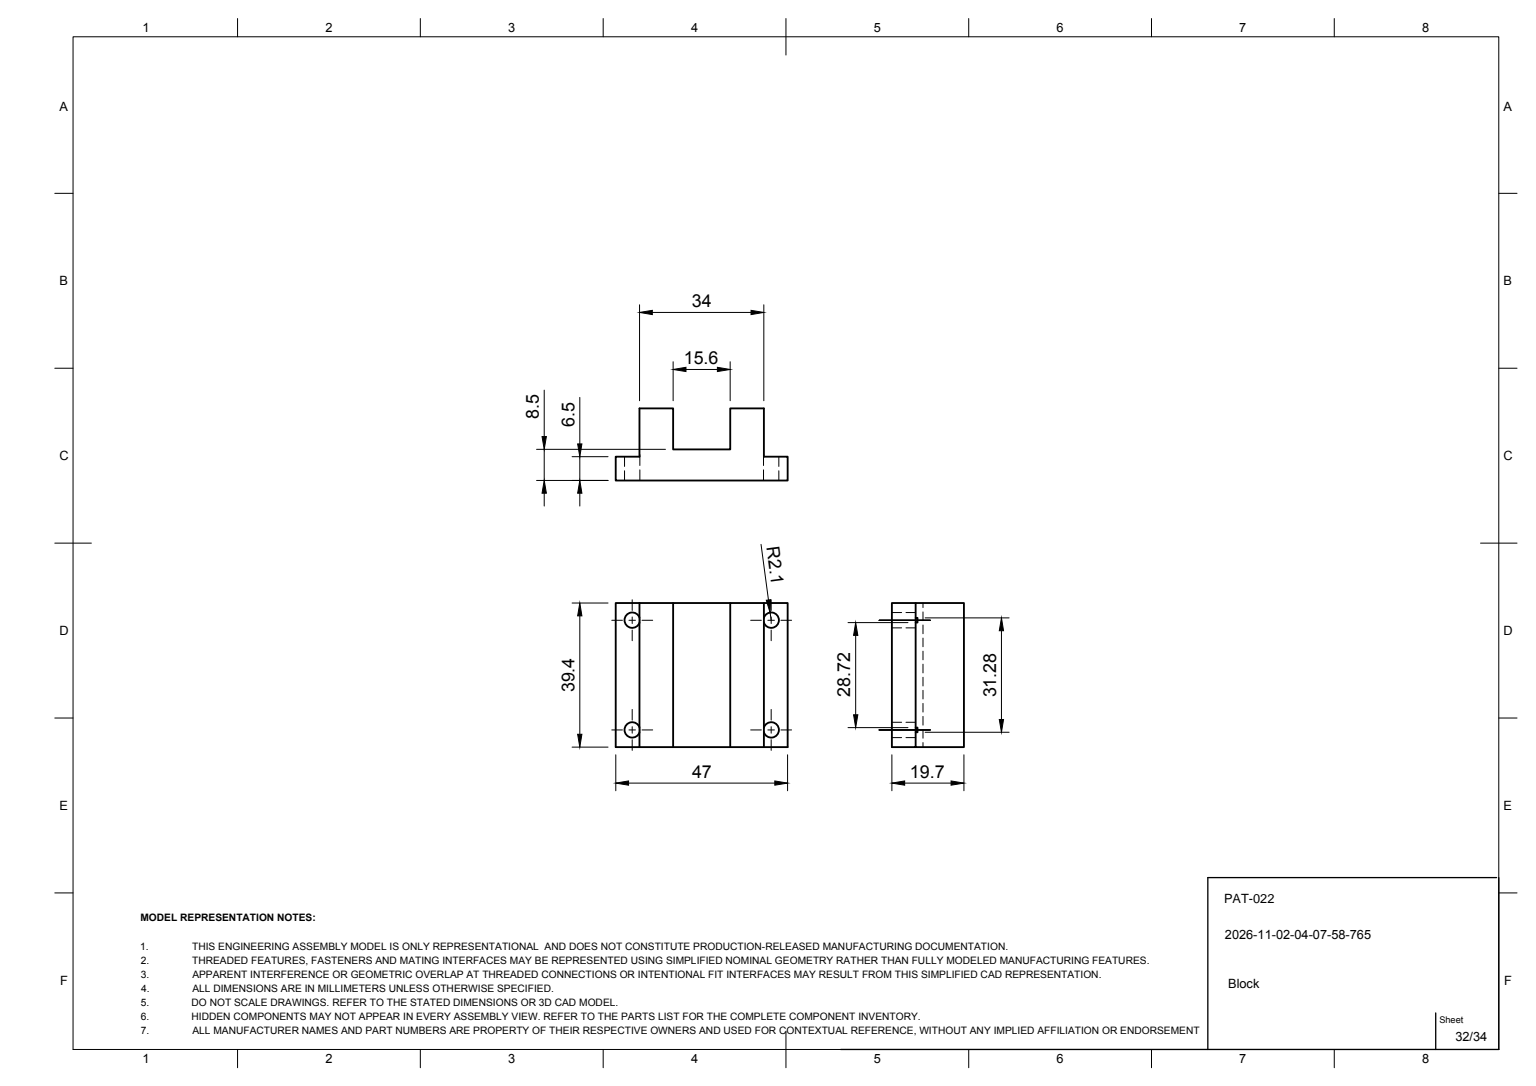
ISO-10303-21;
HEADER;
/* Generated by software containing ST-Developer
 * from STEP Tools, Inc. (www.steptools.com) 
 */

FILE_DESCRIPTION(
/* description */ ('Chute with adjustable gate'),
/* implementation_level */ '2;1');

FILE_NAME(
/* name */ 'Block.step',
/* time_stamp */ '2026-10-27T10:52:28-07:00',
/* author */ (''),
/* organization */ (''),
/* preprocessor_version */ 'ST-DEVELOPER v20.2',
/* originating_system */ 'Autodesk Translation Framework v15.17.0.0',
/* authorisation */ '');

FILE_SCHEMA (('AUTOMOTIVE_DESIGN { 1 0 10303 214 3 1 1 }'));
ENDSEC;

DATA;
#10=MECHANICAL_DESIGN_GEOMETRIC_PRESENTATION_REPRESENTATION('',(#441),#13094);
#377=SHAPE_REPRESENTATION_RELATIONSHIP('SRR','None',#13280,#409);
#409=ADVANCED_BREP_SHAPE_REPRESENTATION('',(#471),#13089);
#441=STYLED_ITEM('',(#13474),#471);
#471=MANIFOLD_SOLID_BREP('Body1',#7626);
#584=FACE_BOUND('',#1793,.T.);
#585=FACE_BOUND('',#1794,.T.);
#586=FACE_BOUND('',#1795,.T.);
#587=FACE_BOUND('',#1796,.T.);
#854=PLANE('',#8510);
#855=PLANE('',#8516);
#856=PLANE('',#8522);
#857=PLANE('',#8528);
#858=PLANE('',#8534);
#859=PLANE('',#8535);
#860=PLANE('',#8536);
#861=PLANE('',#8537);
#862=PLANE('',#8538);
#863=PLANE('',#8539);
#864=PLANE('',#8540);
#865=PLANE('',#8541);
#866=PLANE('',#8542);
#867=PLANE('',#8543);
#868=PLANE('',#8544);
#869=PLANE('',#8545);
#870=PLANE('',#8546);
#871=PLANE('',#8547);
#1254=FACE_OUTER_BOUND('',#1779,.T.);
#1255=FACE_OUTER_BOUND('',#1780,.T.);
#1256=FACE_OUTER_BOUND('',#1781,.T.);
#1257=FACE_OUTER_BOUND('',#1782,.T.);
#1258=FACE_OUTER_BOUND('',#1783,.T.);
#1259=FACE_OUTER_BOUND('',#1784,.T.);
#1260=FACE_OUTER_BOUND('',#1785,.T.);
#1261=FACE_OUTER_BOUND('',#1786,.T.);
#1262=FACE_OUTER_BOUND('',#1787,.T.);
#1263=FACE_OUTER_BOUND('',#1788,.T.);
#1264=FACE_OUTER_BOUND('',#1789,.T.);
#1265=FACE_OUTER_BOUND('',#1790,.T.);
#1266=FACE_OUTER_BOUND('',#1791,.T.);
#1267=FACE_OUTER_BOUND('',#1792,.T.);
#1268=FACE_OUTER_BOUND('',#1797,.T.);
#1269=FACE_OUTER_BOUND('',#1798,.T.);
#1270=FACE_OUTER_BOUND('',#1799,.T.);
#1271=FACE_OUTER_BOUND('',#1800,.T.);
#1272=FACE_OUTER_BOUND('',#1801,.T.);
#1273=FACE_OUTER_BOUND('',#1802,.T.);
#1274=FACE_OUTER_BOUND('',#1803,.T.);
#1275=FACE_OUTER_BOUND('',#1804,.T.);
#1779=EDGE_LOOP('',(#6742,#6743));
#1780=EDGE_LOOP('',(#6744,#6745,#6746,#6747,#6748,#6749,#6750,#6751));
#1781=EDGE_LOOP('',(#6752,#6753));
#1782=EDGE_LOOP('',(#6754,#6755,#6756,#6757,#6758,#6759,#6760,#6761));
#1783=EDGE_LOOP('',(#6762,#6763));
#1784=EDGE_LOOP('',(#6764,#6765,#6766,#6767,#6768,#6769,#6770,#6771));
#1785=EDGE_LOOP('',(#6772,#6773));
#1786=EDGE_LOOP('',(#6774,#6775,#6776,#6777,#6778,#6779,#6780,#6781));
#1787=EDGE_LOOP('',(#6782,#6783,#6784,#6785,#6786,#6787,#6788,#6789,#6790,
#6791,#6792,#6793));
#1788=EDGE_LOOP('',(#6794,#6795,#6796,#6797,#6798,#6799,#6800,#6801,#6802,
#6803,#6804,#6805));
#1789=EDGE_LOOP('',(#6806,#6807,#6808,#6809,#6810,#6811,#6812,#6813,#6814,
#6815,#6816,#6817));
#1790=EDGE_LOOP('',(#6818,#6819,#6820,#6821,#6822,#6823,#6824,#6825,#6826,
#6827));
#1791=EDGE_LOOP('',(#6828,#6829,#6830,#6831));
#1792=EDGE_LOOP('',(#6832,#6833,#6834,#6835));
#1793=EDGE_LOOP('',(#6836));
#1794=EDGE_LOOP('',(#6837));
#1795=EDGE_LOOP('',(#6838));
#1796=EDGE_LOOP('',(#6839));
#1797=EDGE_LOOP('',(#6840,#6841,#6842,#6843));
#1798=EDGE_LOOP('',(#6844,#6845,#6846,#6847,#6848,#6849,#6850,#6851,#6852,
#6853));
#1799=EDGE_LOOP('',(#6854,#6855,#6856,#6857));
#1800=EDGE_LOOP('',(#6858,#6859,#6860,#6861));
#1801=EDGE_LOOP('',(#6862,#6863,#6864,#6865));
#1802=EDGE_LOOP('',(#6866,#6867,#6868,#6869));
#1803=EDGE_LOOP('',(#6870,#6871,#6872,#6873));
#1804=EDGE_LOOP('',(#6874,#6875,#6876,#6877,#6878,#6879,#6880,#6881,#6882,
#6883,#6884,#6885));
#2486=LINE('',#12566,#3263);
#2487=LINE('',#12570,#3264);
#2488=LINE('',#12574,#3265);
#2489=LINE('',#12578,#3266);
#2490=LINE('',#12582,#3267);
#2491=LINE('',#12586,#3268);
#2492=LINE('',#12590,#3269);
#2493=LINE('',#12594,#3270);
#2494=LINE('',#12598,#3271);
#2495=LINE('',#12602,#3272);
#2496=LINE('',#12606,#3273);
#2497=LINE('',#12610,#3274);
#2498=LINE('',#12614,#3275);
#2499=LINE('',#12618,#3276);
#2500=LINE('',#12622,#3277);
#2501=LINE('',#12626,#3278);
#2502=LINE('',#12628,#3279);
#2503=LINE('',#12630,#3280);
#2504=LINE('',#12632,#3281);
#2505=LINE('',#12634,#3282);
#2506=LINE('',#12636,#3283);
#2507=LINE('',#12637,#3284);
#2508=LINE('',#12639,#3285);
#2509=LINE('',#12641,#3286);
#2510=LINE('',#12643,#3287);
#2511=LINE('',#12645,#3288);
#2512=LINE('',#12647,#3289);
#2513=LINE('',#12648,#3290);
#2514=LINE('',#12651,#3291);
#2515=LINE('',#12653,#3292);
#2516=LINE('',#12655,#3293);
#2517=LINE('',#12657,#3294);
#2518=LINE('',#12658,#3295);
#2519=LINE('',#12660,#3296);
#2520=LINE('',#12662,#3297);
#2521=LINE('',#12664,#3298);
#2522=LINE('',#12666,#3299);
#2523=LINE('',#12667,#3300);
#2524=LINE('',#12670,#3301);
#2525=LINE('',#12671,#3302);
#2526=LINE('',#12674,#3303);
#2527=LINE('',#12675,#3304);
#2528=LINE('',#12678,#3305);
#2529=LINE('',#12679,#3306);
#2530=LINE('',#12682,#3307);
#2531=LINE('',#12683,#3308);
#2532=LINE('',#12685,#3309);
#2533=LINE('',#12688,#3310);
#2534=LINE('',#12689,#3311);
#2535=LINE('',#12692,#3312);
#2536=LINE('',#12693,#3313);
#2537=LINE('',#12696,#3314);
#2538=LINE('',#12697,#3315);
#2539=LINE('',#12700,#3316);
#2540=LINE('',#12701,#3317);
#2541=LINE('',#12703,#3318);
#3263=VECTOR('',#10374,1.);
#3264=VECTOR('',#10379,1.);
#3265=VECTOR('',#10382,0.21);
#3266=VECTOR('',#10387,1.);
#3267=VECTOR('',#10390,1.);
#3268=VECTOR('',#10395,1.);
#3269=VECTOR('',#10398,0.21);
#3270=VECTOR('',#10403,1.);
#3271=VECTOR('',#10406,1.);
#3272=VECTOR('',#10411,1.);
#3273=VECTOR('',#10414,0.21);
#3274=VECTOR('',#10419,1.);
#3275=VECTOR('',#10422,1.);
#3276=VECTOR('',#10427,1.);
#3277=VECTOR('',#10430,0.21);
#3278=VECTOR('',#10435,1.);
#3279=VECTOR('',#10438,1.);
#3280=VECTOR('',#10439,1.);
#3281=VECTOR('',#10440,1.);
#3282=VECTOR('',#10441,1.);
#3283=VECTOR('',#10442,1.);
#3284=VECTOR('',#10443,1.);
#3285=VECTOR('',#10446,1.);
#3286=VECTOR('',#10447,1.);
#3287=VECTOR('',#10448,1.);
#3288=VECTOR('',#10449,1.);
#3289=VECTOR('',#10450,1.);
#3290=VECTOR('',#10451,1.);
#3291=VECTOR('',#10454,1.);
#3292=VECTOR('',#10455,1.);
#3293=VECTOR('',#10456,1.);
#3294=VECTOR('',#10457,1.);
#3295=VECTOR('',#10458,1.);
#3296=VECTOR('',#10459,1.);
#3297=VECTOR('',#10460,1.);
#3298=VECTOR('',#10461,1.);
#3299=VECTOR('',#10462,1.);
#3300=VECTOR('',#10463,1.);
#3301=VECTOR('',#10466,1.);
#3302=VECTOR('',#10467,1.);
#3303=VECTOR('',#10470,1.);
#3304=VECTOR('',#10471,1.);
#3305=VECTOR('',#10474,1.);
#3306=VECTOR('',#10475,1.);
#3307=VECTOR('',#10478,1.);
#3308=VECTOR('',#10479,1.);
#3309=VECTOR('',#10482,1.);
#3310=VECTOR('',#10485,1.);
#3311=VECTOR('',#10486,1.);
#3312=VECTOR('',#10489,1.);
#3313=VECTOR('',#10490,1.);
#3314=VECTOR('',#10493,1.);
#3315=VECTOR('',#10494,1.);
#3316=VECTOR('',#10497,1.);
#3317=VECTOR('',#10498,1.);
#3318=VECTOR('',#10501,1.);
#3562=CIRCLE('',#8511,0.21);
#3563=CIRCLE('',#8513,0.21);
#3564=CIRCLE('',#8514,0.21);
#3565=CIRCLE('',#8515,0.21);
#3566=CIRCLE('',#8517,0.21);
#3567=CIRCLE('',#8519,0.21);
#3568=CIRCLE('',#8520,0.21);
#3569=CIRCLE('',#8521,0.21);
#3570=CIRCLE('',#8523,0.21);
#3571=CIRCLE('',#8525,0.21);
#3572=CIRCLE('',#8526,0.21);
#3573=CIRCLE('',#8527,0.21);
#3574=CIRCLE('',#8529,0.21);
#3575=CIRCLE('',#8531,0.21);
#3576=CIRCLE('',#8532,0.21);
#3577=CIRCLE('',#8533,0.21);
#4107=VERTEX_POINT('',#12564);
#4108=VERTEX_POINT('',#12565);
#4109=VERTEX_POINT('',#12569);
#4110=VERTEX_POINT('',#12571);
#4111=VERTEX_POINT('',#12573);
#4112=VERTEX_POINT('',#12576);
#4113=VERTEX_POINT('',#12580);
#4114=VERTEX_POINT('',#12581);
#4115=VERTEX_POINT('',#12585);
#4116=VERTEX_POINT('',#12587);
#4117=VERTEX_POINT('',#12589);
#4118=VERTEX_POINT('',#12592);
#4119=VERTEX_POINT('',#12596);
#4120=VERTEX_POINT('',#12597);
#4121=VERTEX_POINT('',#12601);
#4122=VERTEX_POINT('',#12603);
#4123=VERTEX_POINT('',#12605);
#4124=VERTEX_POINT('',#12608);
#4125=VERTEX_POINT('',#12612);
#4126=VERTEX_POINT('',#12613);
#4127=VERTEX_POINT('',#12617);
#4128=VERTEX_POINT('',#12619);
#4129=VERTEX_POINT('',#12621);
#4130=VERTEX_POINT('',#12624);
#4131=VERTEX_POINT('',#12629);
#4132=VERTEX_POINT('',#12631);
#4133=VERTEX_POINT('',#12633);
#4134=VERTEX_POINT('',#12635);
#4135=VERTEX_POINT('',#12640);
#4136=VERTEX_POINT('',#12642);
#4137=VERTEX_POINT('',#12644);
#4138=VERTEX_POINT('',#12646);
#4139=VERTEX_POINT('',#12650);
#4140=VERTEX_POINT('',#12652);
#4141=VERTEX_POINT('',#12654);
#4142=VERTEX_POINT('',#12656);
#4143=VERTEX_POINT('',#12659);
#4144=VERTEX_POINT('',#12661);
#4145=VERTEX_POINT('',#12663);
#4146=VERTEX_POINT('',#12665);
#4147=VERTEX_POINT('',#12669);
#4148=VERTEX_POINT('',#12673);
#4149=VERTEX_POINT('',#12677);
#4150=VERTEX_POINT('',#12681);
#4151=VERTEX_POINT('',#12687);
#4152=VERTEX_POINT('',#12691);
#4153=VERTEX_POINT('',#12695);
#4154=VERTEX_POINT('',#12699);
#5004=EDGE_CURVE('',#4107,#4108,#2486,.T.);
#5005=EDGE_CURVE('',#4107,#4108,#3562,.T.);
#5006=EDGE_CURVE('',#4109,#4107,#2487,.T.);
#5007=EDGE_CURVE('',#4110,#4109,#3563,.T.);
#5008=EDGE_CURVE('',#4110,#4111,#2488,.T.);
#5009=EDGE_CURVE('',#4111,#4111,#3564,.T.);
#5010=EDGE_CURVE('',#4112,#4110,#3565,.T.);
#5011=EDGE_CURVE('',#4108,#4112,#2489,.T.);
#5012=EDGE_CURVE('',#4113,#4114,#2490,.T.);
#5013=EDGE_CURVE('',#4113,#4114,#3566,.T.);
#5014=EDGE_CURVE('',#4115,#4113,#2491,.T.);
#5015=EDGE_CURVE('',#4116,#4115,#3567,.T.);
#5016=EDGE_CURVE('',#4116,#4117,#2492,.T.);
#5017=EDGE_CURVE('',#4117,#4117,#3568,.T.);
#5018=EDGE_CURVE('',#4118,#4116,#3569,.T.);
#5019=EDGE_CURVE('',#4114,#4118,#2493,.T.);
#5020=EDGE_CURVE('',#4119,#4120,#2494,.T.);
#5021=EDGE_CURVE('',#4119,#4120,#3570,.T.);
#5022=EDGE_CURVE('',#4121,#4119,#2495,.T.);
#5023=EDGE_CURVE('',#4122,#4121,#3571,.T.);
#5024=EDGE_CURVE('',#4122,#4123,#2496,.T.);
#5025=EDGE_CURVE('',#4123,#4123,#3572,.T.);
#5026=EDGE_CURVE('',#4124,#4122,#3573,.T.);
#5027=EDGE_CURVE('',#4120,#4124,#2497,.T.);
#5028=EDGE_CURVE('',#4125,#4126,#2498,.T.);
#5029=EDGE_CURVE('',#4125,#4126,#3574,.T.);
#5030=EDGE_CURVE('',#4127,#4125,#2499,.T.);
#5031=EDGE_CURVE('',#4128,#4127,#3575,.T.);
#5032=EDGE_CURVE('',#4128,#4129,#2500,.T.);
#5033=EDGE_CURVE('',#4129,#4129,#3576,.T.);
#5034=EDGE_CURVE('',#4130,#4128,#3577,.T.);
#5035=EDGE_CURVE('',#4126,#4130,#2501,.T.);
#5036=EDGE_CURVE('',#4112,#4121,#2502,.T.);
#5037=EDGE_CURVE('',#4124,#4131,#2503,.T.);
#5038=EDGE_CURVE('',#4132,#4131,#2504,.T.);
#5039=EDGE_CURVE('',#4132,#4133,#2505,.T.);
#5040=EDGE_CURVE('',#4134,#4133,#2506,.T.);
#5041=EDGE_CURVE('',#4134,#4109,#2507,.T.);
#5042=EDGE_CURVE('',#4118,#4127,#2508,.T.);
#5043=EDGE_CURVE('',#4130,#4135,#2509,.T.);
#5044=EDGE_CURVE('',#4136,#4135,#2510,.T.);
#5045=EDGE_CURVE('',#4137,#4136,#2511,.T.);
#5046=EDGE_CURVE('',#4138,#4137,#2512,.T.);
#5047=EDGE_CURVE('',#4138,#4115,#2513,.T.);
#5048=EDGE_CURVE('',#4131,#4139,#2514,.T.);
#5049=EDGE_CURVE('',#4139,#4140,#2515,.T.);
#5050=EDGE_CURVE('',#4140,#4141,#2516,.T.);
#5051=EDGE_CURVE('',#4141,#4142,#2517,.T.);
#5052=EDGE_CURVE('',#4142,#4138,#2518,.T.);
#5053=EDGE_CURVE('',#4137,#4143,#2519,.T.);
#5054=EDGE_CURVE('',#4143,#4144,#2520,.T.);
#5055=EDGE_CURVE('',#4144,#4145,#2521,.T.);
#5056=EDGE_CURVE('',#4145,#4146,#2522,.T.);
#5057=EDGE_CURVE('',#4146,#4132,#2523,.T.);
#5058=EDGE_CURVE('',#4147,#4134,#2524,.T.);
#5059=EDGE_CURVE('',#4139,#4147,#2525,.T.);
#5060=EDGE_CURVE('',#4148,#4147,#2526,.T.);
#5061=EDGE_CURVE('',#4140,#4148,#2527,.T.);
#5062=EDGE_CURVE('',#4149,#4148,#2528,.T.);
#5063=EDGE_CURVE('',#4141,#4149,#2529,.T.);
#5064=EDGE_CURVE('',#4150,#4149,#2530,.T.);
#5065=EDGE_CURVE('',#4142,#4150,#2531,.T.);
#5066=EDGE_CURVE('',#4135,#4150,#2532,.T.);
#5067=EDGE_CURVE('',#4151,#4136,#2533,.T.);
#5068=EDGE_CURVE('',#4143,#4151,#2534,.T.);
#5069=EDGE_CURVE('',#4152,#4151,#2535,.T.);
#5070=EDGE_CURVE('',#4144,#4152,#2536,.T.);
#5071=EDGE_CURVE('',#4153,#4152,#2537,.T.);
#5072=EDGE_CURVE('',#4145,#4153,#2538,.T.);
#5073=EDGE_CURVE('',#4154,#4153,#2539,.T.);
#5074=EDGE_CURVE('',#4146,#4154,#2540,.T.);
#5075=EDGE_CURVE('',#4133,#4154,#2541,.T.);
#6742=ORIENTED_EDGE('',*,*,#5004,.F.);
#6743=ORIENTED_EDGE('',*,*,#5005,.T.);
#6744=ORIENTED_EDGE('',*,*,#5006,.F.);
#6745=ORIENTED_EDGE('',*,*,#5007,.F.);
#6746=ORIENTED_EDGE('',*,*,#5008,.T.);
#6747=ORIENTED_EDGE('',*,*,#5009,.F.);
#6748=ORIENTED_EDGE('',*,*,#5008,.F.);
#6749=ORIENTED_EDGE('',*,*,#5010,.F.);
#6750=ORIENTED_EDGE('',*,*,#5011,.F.);
#6751=ORIENTED_EDGE('',*,*,#5005,.F.);
#6752=ORIENTED_EDGE('',*,*,#5012,.F.);
#6753=ORIENTED_EDGE('',*,*,#5013,.T.);
#6754=ORIENTED_EDGE('',*,*,#5014,.F.);
#6755=ORIENTED_EDGE('',*,*,#5015,.F.);
#6756=ORIENTED_EDGE('',*,*,#5016,.T.);
#6757=ORIENTED_EDGE('',*,*,#5017,.F.);
#6758=ORIENTED_EDGE('',*,*,#5016,.F.);
#6759=ORIENTED_EDGE('',*,*,#5018,.F.);
#6760=ORIENTED_EDGE('',*,*,#5019,.F.);
#6761=ORIENTED_EDGE('',*,*,#5013,.F.);
#6762=ORIENTED_EDGE('',*,*,#5020,.F.);
#6763=ORIENTED_EDGE('',*,*,#5021,.T.);
#6764=ORIENTED_EDGE('',*,*,#5022,.F.);
#6765=ORIENTED_EDGE('',*,*,#5023,.F.);
#6766=ORIENTED_EDGE('',*,*,#5024,.T.);
#6767=ORIENTED_EDGE('',*,*,#5025,.F.);
#6768=ORIENTED_EDGE('',*,*,#5024,.F.);
#6769=ORIENTED_EDGE('',*,*,#5026,.F.);
#6770=ORIENTED_EDGE('',*,*,#5027,.F.);
#6771=ORIENTED_EDGE('',*,*,#5021,.F.);
#6772=ORIENTED_EDGE('',*,*,#5028,.F.);
#6773=ORIENTED_EDGE('',*,*,#5029,.T.);
#6774=ORIENTED_EDGE('',*,*,#5030,.F.);
#6775=ORIENTED_EDGE('',*,*,#5031,.F.);
#6776=ORIENTED_EDGE('',*,*,#5032,.T.);
#6777=ORIENTED_EDGE('',*,*,#5033,.F.);
#6778=ORIENTED_EDGE('',*,*,#5032,.F.);
#6779=ORIENTED_EDGE('',*,*,#5034,.F.);
#6780=ORIENTED_EDGE('',*,*,#5035,.F.);
#6781=ORIENTED_EDGE('',*,*,#5029,.F.);
#6782=ORIENTED_EDGE('',*,*,#5006,.T.);
#6783=ORIENTED_EDGE('',*,*,#5004,.T.);
#6784=ORIENTED_EDGE('',*,*,#5011,.T.);
#6785=ORIENTED_EDGE('',*,*,#5036,.T.);
#6786=ORIENTED_EDGE('',*,*,#5022,.T.);
#6787=ORIENTED_EDGE('',*,*,#5020,.T.);
#6788=ORIENTED_EDGE('',*,*,#5027,.T.);
#6789=ORIENTED_EDGE('',*,*,#5037,.T.);
#6790=ORIENTED_EDGE('',*,*,#5038,.F.);
#6791=ORIENTED_EDGE('',*,*,#5039,.T.);
#6792=ORIENTED_EDGE('',*,*,#5040,.F.);
#6793=ORIENTED_EDGE('',*,*,#5041,.T.);
#6794=ORIENTED_EDGE('',*,*,#5014,.T.);
#6795=ORIENTED_EDGE('',*,*,#5012,.T.);
#6796=ORIENTED_EDGE('',*,*,#5019,.T.);
#6797=ORIENTED_EDGE('',*,*,#5042,.T.);
#6798=ORIENTED_EDGE('',*,*,#5030,.T.);
#6799=ORIENTED_EDGE('',*,*,#5028,.T.);
#6800=ORIENTED_EDGE('',*,*,#5035,.T.);
#6801=ORIENTED_EDGE('',*,*,#5043,.T.);
#6802=ORIENTED_EDGE('',*,*,#5044,.F.);
#6803=ORIENTED_EDGE('',*,*,#5045,.F.);
#6804=ORIENTED_EDGE('',*,*,#5046,.F.);
#6805=ORIENTED_EDGE('',*,*,#5047,.T.);
#6806=ORIENTED_EDGE('',*,*,#5038,.T.);
#6807=ORIENTED_EDGE('',*,*,#5048,.T.);
#6808=ORIENTED_EDGE('',*,*,#5049,.T.);
#6809=ORIENTED_EDGE('',*,*,#5050,.T.);
#6810=ORIENTED_EDGE('',*,*,#5051,.T.);
#6811=ORIENTED_EDGE('',*,*,#5052,.T.);
#6812=ORIENTED_EDGE('',*,*,#5046,.T.);
#6813=ORIENTED_EDGE('',*,*,#5053,.T.);
#6814=ORIENTED_EDGE('',*,*,#5054,.T.);
#6815=ORIENTED_EDGE('',*,*,#5055,.T.);
#6816=ORIENTED_EDGE('',*,*,#5056,.T.);
#6817=ORIENTED_EDGE('',*,*,#5057,.T.);
#6818=ORIENTED_EDGE('',*,*,#5010,.T.);
#6819=ORIENTED_EDGE('',*,*,#5007,.T.);
#6820=ORIENTED_EDGE('',*,*,#5041,.F.);
#6821=ORIENTED_EDGE('',*,*,#5058,.F.);
#6822=ORIENTED_EDGE('',*,*,#5059,.F.);
#6823=ORIENTED_EDGE('',*,*,#5048,.F.);
#6824=ORIENTED_EDGE('',*,*,#5037,.F.);
#6825=ORIENTED_EDGE('',*,*,#5026,.T.);
#6826=ORIENTED_EDGE('',*,*,#5023,.T.);
#6827=ORIENTED_EDGE('',*,*,#5036,.F.);
#6828=ORIENTED_EDGE('',*,*,#5059,.T.);
#6829=ORIENTED_EDGE('',*,*,#5060,.F.);
#6830=ORIENTED_EDGE('',*,*,#5061,.F.);
#6831=ORIENTED_EDGE('',*,*,#5049,.F.);
#6832=ORIENTED_EDGE('',*,*,#5061,.T.);
#6833=ORIENTED_EDGE('',*,*,#5062,.F.);
#6834=ORIENTED_EDGE('',*,*,#5063,.F.);
#6835=ORIENTED_EDGE('',*,*,#5050,.F.);
#6836=ORIENTED_EDGE('',*,*,#5009,.T.);
#6837=ORIENTED_EDGE('',*,*,#5017,.T.);
#6838=ORIENTED_EDGE('',*,*,#5025,.T.);
#6839=ORIENTED_EDGE('',*,*,#5033,.T.);
#6840=ORIENTED_EDGE('',*,*,#5063,.T.);
#6841=ORIENTED_EDGE('',*,*,#5064,.F.);
#6842=ORIENTED_EDGE('',*,*,#5065,.F.);
#6843=ORIENTED_EDGE('',*,*,#5051,.F.);
#6844=ORIENTED_EDGE('',*,*,#5018,.T.);
#6845=ORIENTED_EDGE('',*,*,#5015,.T.);
#6846=ORIENTED_EDGE('',*,*,#5047,.F.);
#6847=ORIENTED_EDGE('',*,*,#5052,.F.);
#6848=ORIENTED_EDGE('',*,*,#5065,.T.);
#6849=ORIENTED_EDGE('',*,*,#5066,.F.);
#6850=ORIENTED_EDGE('',*,*,#5043,.F.);
#6851=ORIENTED_EDGE('',*,*,#5034,.T.);
#6852=ORIENTED_EDGE('',*,*,#5031,.T.);
#6853=ORIENTED_EDGE('',*,*,#5042,.F.);
#6854=ORIENTED_EDGE('',*,*,#5045,.T.);
#6855=ORIENTED_EDGE('',*,*,#5067,.F.);
#6856=ORIENTED_EDGE('',*,*,#5068,.F.);
#6857=ORIENTED_EDGE('',*,*,#5053,.F.);
#6858=ORIENTED_EDGE('',*,*,#5068,.T.);
#6859=ORIENTED_EDGE('',*,*,#5069,.F.);
#6860=ORIENTED_EDGE('',*,*,#5070,.F.);
#6861=ORIENTED_EDGE('',*,*,#5054,.F.);
#6862=ORIENTED_EDGE('',*,*,#5070,.T.);
#6863=ORIENTED_EDGE('',*,*,#5071,.F.);
#6864=ORIENTED_EDGE('',*,*,#5072,.F.);
#6865=ORIENTED_EDGE('',*,*,#5055,.F.);
#6866=ORIENTED_EDGE('',*,*,#5072,.T.);
#6867=ORIENTED_EDGE('',*,*,#5073,.F.);
#6868=ORIENTED_EDGE('',*,*,#5074,.F.);
#6869=ORIENTED_EDGE('',*,*,#5056,.F.);
#6870=ORIENTED_EDGE('',*,*,#5074,.T.);
#6871=ORIENTED_EDGE('',*,*,#5075,.F.);
#6872=ORIENTED_EDGE('',*,*,#5039,.F.);
#6873=ORIENTED_EDGE('',*,*,#5057,.F.);
#6874=ORIENTED_EDGE('',*,*,#5040,.T.);
#6875=ORIENTED_EDGE('',*,*,#5075,.T.);
#6876=ORIENTED_EDGE('',*,*,#5073,.T.);
#6877=ORIENTED_EDGE('',*,*,#5071,.T.);
#6878=ORIENTED_EDGE('',*,*,#5069,.T.);
#6879=ORIENTED_EDGE('',*,*,#5067,.T.);
#6880=ORIENTED_EDGE('',*,*,#5044,.T.);
#6881=ORIENTED_EDGE('',*,*,#5066,.T.);
#6882=ORIENTED_EDGE('',*,*,#5064,.T.);
#6883=ORIENTED_EDGE('',*,*,#5062,.T.);
#6884=ORIENTED_EDGE('',*,*,#5060,.T.);
#6885=ORIENTED_EDGE('',*,*,#5058,.T.);
#7174=CYLINDRICAL_SURFACE('',#8512,0.21);
#7175=CYLINDRICAL_SURFACE('',#8518,0.21);
#7176=CYLINDRICAL_SURFACE('',#8524,0.21);
#7177=CYLINDRICAL_SURFACE('',#8530,0.21);
#7522=ADVANCED_FACE('',(#1254),#854,.T.);
#7523=ADVANCED_FACE('',(#1255),#7174,.F.);
#7524=ADVANCED_FACE('',(#1256),#855,.T.);
#7525=ADVANCED_FACE('',(#1257),#7175,.F.);
#7526=ADVANCED_FACE('',(#1258),#856,.T.);
#7527=ADVANCED_FACE('',(#1259),#7176,.F.);
#7528=ADVANCED_FACE('',(#1260),#857,.T.);
#7529=ADVANCED_FACE('',(#1261),#7177,.F.);
#7530=ADVANCED_FACE('',(#1262),#858,.T.);
#7531=ADVANCED_FACE('',(#1263),#859,.T.);
#7532=ADVANCED_FACE('',(#1264),#860,.T.);
#7533=ADVANCED_FACE('',(#1265),#861,.T.);
#7534=ADVANCED_FACE('',(#1266),#862,.T.);
#7535=ADVANCED_FACE('',(#1267,#584,#585,#586,#587),#863,.T.);
#7536=ADVANCED_FACE('',(#1268),#864,.T.);
#7537=ADVANCED_FACE('',(#1269),#865,.T.);
#7538=ADVANCED_FACE('',(#1270),#866,.T.);
#7539=ADVANCED_FACE('',(#1271),#867,.T.);
#7540=ADVANCED_FACE('',(#1272),#868,.T.);
#7541=ADVANCED_FACE('',(#1273),#869,.T.);
#7542=ADVANCED_FACE('',(#1274),#870,.T.);
#7543=ADVANCED_FACE('',(#1275),#871,.T.);
#7626=CLOSED_SHELL('',(#7522,#7523,#7524,#7525,#7526,#7527,#7528,#7529,
#7530,#7531,#7532,#7533,#7534,#7535,#7536,#7537,#7538,#7539,#7540,#7541,
#7542,#7543));
#8509=AXIS2_PLACEMENT_3D('',#12562,#10370,#10371);
#8510=AXIS2_PLACEMENT_3D('',#12563,#10372,#10373);
#8511=AXIS2_PLACEMENT_3D('',#12567,#10375,#10376);
#8512=AXIS2_PLACEMENT_3D('',#12568,#10377,#10378);
#8513=AXIS2_PLACEMENT_3D('',#12572,#10380,#10381);
#8514=AXIS2_PLACEMENT_3D('',#12575,#10383,#10384);
#8515=AXIS2_PLACEMENT_3D('',#12577,#10385,#10386);
#8516=AXIS2_PLACEMENT_3D('',#12579,#10388,#10389);
#8517=AXIS2_PLACEMENT_3D('',#12583,#10391,#10392);
#8518=AXIS2_PLACEMENT_3D('',#12584,#10393,#10394);
#8519=AXIS2_PLACEMENT_3D('',#12588,#10396,#10397);
#8520=AXIS2_PLACEMENT_3D('',#12591,#10399,#10400);
#8521=AXIS2_PLACEMENT_3D('',#12593,#10401,#10402);
#8522=AXIS2_PLACEMENT_3D('',#12595,#10404,#10405);
#8523=AXIS2_PLACEMENT_3D('',#12599,#10407,#10408);
#8524=AXIS2_PLACEMENT_3D('',#12600,#10409,#10410);
#8525=AXIS2_PLACEMENT_3D('',#12604,#10412,#10413);
#8526=AXIS2_PLACEMENT_3D('',#12607,#10415,#10416);
#8527=AXIS2_PLACEMENT_3D('',#12609,#10417,#10418);
#8528=AXIS2_PLACEMENT_3D('',#12611,#10420,#10421);
#8529=AXIS2_PLACEMENT_3D('',#12615,#10423,#10424);
#8530=AXIS2_PLACEMENT_3D('',#12616,#10425,#10426);
#8531=AXIS2_PLACEMENT_3D('',#12620,#10428,#10429);
#8532=AXIS2_PLACEMENT_3D('',#12623,#10431,#10432);
#8533=AXIS2_PLACEMENT_3D('',#12625,#10433,#10434);
#8534=AXIS2_PLACEMENT_3D('',#12627,#10436,#10437);
#8535=AXIS2_PLACEMENT_3D('',#12638,#10444,#10445);
#8536=AXIS2_PLACEMENT_3D('',#12649,#10452,#10453);
#8537=AXIS2_PLACEMENT_3D('',#12668,#10464,#10465);
#8538=AXIS2_PLACEMENT_3D('',#12672,#10468,#10469);
#8539=AXIS2_PLACEMENT_3D('',#12676,#10472,#10473);
#8540=AXIS2_PLACEMENT_3D('',#12680,#10476,#10477);
#8541=AXIS2_PLACEMENT_3D('',#12684,#10480,#10481);
#8542=AXIS2_PLACEMENT_3D('',#12686,#10483,#10484);
#8543=AXIS2_PLACEMENT_3D('',#12690,#10487,#10488);
#8544=AXIS2_PLACEMENT_3D('',#12694,#10491,#10492);
#8545=AXIS2_PLACEMENT_3D('',#12698,#10495,#10496);
#8546=AXIS2_PLACEMENT_3D('',#12702,#10499,#10500);
#8547=AXIS2_PLACEMENT_3D('',#12704,#10502,#10503);
#10370=DIRECTION('axis',(0.,0.,1.));
#10371=DIRECTION('refdir',(1.,0.,0.));
#10372=DIRECTION('center_axis',(0.,0.,1.));
#10373=DIRECTION('ref_axis',(1.,0.,0.));
#10374=DIRECTION('',(-1.,0.,0.));
#10375=DIRECTION('center_axis',(0.,0.,1.));
#10376=DIRECTION('ref_axis',(1.,0.,0.));
#10377=DIRECTION('center_axis',(0.,0.,1.));
#10378=DIRECTION('ref_axis',(1.,0.,0.));
#10379=DIRECTION('',(0.,0.,-1.));
#10380=DIRECTION('center_axis',(0.,0.,1.));
#10381=DIRECTION('ref_axis',(1.,0.,0.));
#10382=DIRECTION('',(0.,0.,1.));
#10383=DIRECTION('center_axis',(0.,0.,-1.));
#10384=DIRECTION('ref_axis',(1.,0.,0.));
#10385=DIRECTION('center_axis',(0.,0.,1.));
#10386=DIRECTION('ref_axis',(1.,0.,0.));
#10387=DIRECTION('',(0.,0.,1.));
#10388=DIRECTION('center_axis',(0.,0.,1.));
#10389=DIRECTION('ref_axis',(1.,0.,0.));
#10390=DIRECTION('',(1.,0.,0.));
#10391=DIRECTION('center_axis',(0.,0.,1.));
#10392=DIRECTION('ref_axis',(1.,0.,0.));
#10393=DIRECTION('center_axis',(0.,0.,1.));
#10394=DIRECTION('ref_axis',(1.,0.,0.));
#10395=DIRECTION('',(0.,0.,-1.));
#10396=DIRECTION('center_axis',(0.,0.,1.));
#10397=DIRECTION('ref_axis',(1.,0.,0.));
#10398=DIRECTION('',(0.,0.,1.));
#10399=DIRECTION('center_axis',(0.,0.,-1.));
#10400=DIRECTION('ref_axis',(1.,0.,0.));
#10401=DIRECTION('center_axis',(0.,0.,1.));
#10402=DIRECTION('ref_axis',(1.,0.,0.));
#10403=DIRECTION('',(0.,0.,1.));
#10404=DIRECTION('center_axis',(0.,0.,1.));
#10405=DIRECTION('ref_axis',(1.,0.,0.));
#10406=DIRECTION('',(-1.,0.,0.));
#10407=DIRECTION('center_axis',(0.,0.,1.));
#10408=DIRECTION('ref_axis',(1.,0.,0.));
#10409=DIRECTION('center_axis',(0.,0.,1.));
#10410=DIRECTION('ref_axis',(1.,0.,0.));
#10411=DIRECTION('',(0.,0.,-1.));
#10412=DIRECTION('center_axis',(0.,0.,1.));
#10413=DIRECTION('ref_axis',(1.,0.,0.));
#10414=DIRECTION('',(0.,0.,1.));
#10415=DIRECTION('center_axis',(0.,0.,-1.));
#10416=DIRECTION('ref_axis',(1.,0.,0.));
#10417=DIRECTION('center_axis',(0.,0.,1.));
#10418=DIRECTION('ref_axis',(1.,0.,0.));
#10419=DIRECTION('',(0.,0.,1.));
#10420=DIRECTION('center_axis',(0.,0.,1.));
#10421=DIRECTION('ref_axis',(1.,0.,0.));
#10422=DIRECTION('',(1.,0.,0.));
#10423=DIRECTION('center_axis',(0.,0.,1.));
#10424=DIRECTION('ref_axis',(1.,0.,0.));
#10425=DIRECTION('center_axis',(0.,0.,1.));
#10426=DIRECTION('ref_axis',(1.,0.,0.));
#10427=DIRECTION('',(0.,0.,-1.));
#10428=DIRECTION('center_axis',(0.,0.,1.));
#10429=DIRECTION('ref_axis',(1.,0.,0.));
#10430=DIRECTION('',(0.,0.,1.));
#10431=DIRECTION('center_axis',(0.,0.,-1.));
#10432=DIRECTION('ref_axis',(1.,0.,0.));
#10433=DIRECTION('center_axis',(0.,0.,1.));
#10434=DIRECTION('ref_axis',(1.,0.,0.));
#10435=DIRECTION('',(0.,0.,1.));
#10436=DIRECTION('center_axis',(0.,-1.,0.));
#10437=DIRECTION('ref_axis',(0.,0.,-1.));
#10438=DIRECTION('',(-1.,0.,0.));
#10439=DIRECTION('',(-1.,0.,0.));
#10440=DIRECTION('',(0.,0.,1.));
#10441=DIRECTION('',(1.,0.,0.));
#10442=DIRECTION('',(0.,0.,-1.));
#10443=DIRECTION('',(-1.,0.,0.));
#10444=DIRECTION('center_axis',(0.,1.,0.));
#10445=DIRECTION('ref_axis',(0.,0.,1.));
#10446=DIRECTION('',(1.,0.,0.));
#10447=DIRECTION('',(1.,0.,0.));
#10448=DIRECTION('',(0.,0.,1.));
#10449=DIRECTION('',(1.,0.,0.));
#10450=DIRECTION('',(0.,0.,-1.));
#10451=DIRECTION('',(1.,0.,0.));
#10452=DIRECTION('center_axis',(-1.,0.,0.));
#10453=DIRECTION('ref_axis',(0.,0.,1.));
#10454=DIRECTION('',(0.,-1.,0.));
#10455=DIRECTION('',(0.,0.,1.));
#10456=DIRECTION('',(0.,1.,0.));
#10457=DIRECTION('',(0.,0.,-1.));
#10458=DIRECTION('',(0.,-1.,0.));
#10459=DIRECTION('',(0.,-1.,0.));
#10460=DIRECTION('',(0.,0.,1.));
#10461=DIRECTION('',(0.,-1.,0.));
#10462=DIRECTION('',(0.,0.,-1.));
#10463=DIRECTION('',(0.,-1.,0.));
#10464=DIRECTION('center_axis',(0.,0.,-1.));
#10465=DIRECTION('ref_axis',(0.,1.,0.));
#10466=DIRECTION('',(0.,1.,0.));
#10467=DIRECTION('',(1.,0.,0.));
#10468=DIRECTION('center_axis',(0.,-1.,0.));
#10469=DIRECTION('ref_axis',(0.,0.,-1.));
#10470=DIRECTION('',(0.,0.,-1.));
#10471=DIRECTION('',(1.,0.,0.));
#10472=DIRECTION('center_axis',(0.,0.,1.));
#10473=DIRECTION('ref_axis',(0.,-1.,0.));
#10474=DIRECTION('',(0.,-1.,0.));
#10475=DIRECTION('',(1.,0.,0.));
#10476=DIRECTION('center_axis',(0.,1.,0.));
#10477=DIRECTION('ref_axis',(0.,0.,1.));
#10478=DIRECTION('',(0.,0.,1.));
#10479=DIRECTION('',(1.,0.,0.));
#10480=DIRECTION('center_axis',(0.,0.,-1.));
#10481=DIRECTION('ref_axis',(0.,1.,0.));
#10482=DIRECTION('',(0.,1.,0.));
#10483=DIRECTION('center_axis',(0.,0.,-1.));
#10484=DIRECTION('ref_axis',(0.,1.,0.));
#10485=DIRECTION('',(0.,1.,0.));
#10486=DIRECTION('',(1.,0.,0.));
#10487=DIRECTION('center_axis',(0.,-1.,0.));
#10488=DIRECTION('ref_axis',(0.,0.,-1.));
#10489=DIRECTION('',(0.,0.,-1.));
#10490=DIRECTION('',(1.,0.,0.));
#10491=DIRECTION('center_axis',(0.,0.,-1.));
#10492=DIRECTION('ref_axis',(0.,1.,0.));
#10493=DIRECTION('',(0.,1.,0.));
#10494=DIRECTION('',(1.,0.,0.));
#10495=DIRECTION('center_axis',(0.,1.,0.));
#10496=DIRECTION('ref_axis',(0.,0.,1.));
#10497=DIRECTION('',(0.,0.,1.));
#10498=DIRECTION('',(1.,0.,0.));
#10499=DIRECTION('center_axis',(0.,0.,-1.));
#10500=DIRECTION('ref_axis',(0.,1.,0.));
#10501=DIRECTION('',(0.,1.,0.));
#10502=DIRECTION('center_axis',(1.,0.,0.));
#10503=DIRECTION('ref_axis',(0.,0.,-1.));
#12562=CARTESIAN_POINT('',(0.,0.,0.));
#12563=CARTESIAN_POINT('Origin',(1.5,-1.9,1.7));
#12564=CARTESIAN_POINT('',(1.56403124237433,-1.7,1.7));
#12565=CARTESIAN_POINT('',(1.43596875762567,-1.7,1.7));
#12566=CARTESIAN_POINT('',(0.75,-1.7,1.7));
#12567=CARTESIAN_POINT('Origin',(1.5,-1.9,1.7));
#12568=CARTESIAN_POINT('Origin',(1.5,-1.9,1.7));
#12569=CARTESIAN_POINT('',(1.56403124237433,-1.7,1.75));
#12570=CARTESIAN_POINT('',(1.56403124237433,-1.7,1.7));
#12571=CARTESIAN_POINT('',(1.29,-1.9,1.75));
#12572=CARTESIAN_POINT('Origin',(1.5,-1.9,1.75));
#12573=CARTESIAN_POINT('',(1.29,-1.9,2.4));
#12574=CARTESIAN_POINT('',(1.29,-1.9,1.7));
#12575=CARTESIAN_POINT('Origin',(1.5,-1.9,2.4));
#12576=CARTESIAN_POINT('',(1.43596875762567,-1.7,1.75));
#12577=CARTESIAN_POINT('Origin',(1.5,-1.9,1.75));
#12578=CARTESIAN_POINT('',(1.43596875762567,-1.7,1.7));
#12579=CARTESIAN_POINT('Origin',(-1.5,1.9,1.7));
#12580=CARTESIAN_POINT('',(-1.56403124237433,1.7,1.7));
#12581=CARTESIAN_POINT('',(-1.43596875762567,1.7,1.7));
#12582=CARTESIAN_POINT('',(-0.75,1.7,1.7));
#12583=CARTESIAN_POINT('Origin',(-1.5,1.9,1.7));
#12584=CARTESIAN_POINT('Origin',(-1.5,1.9,1.7));
#12585=CARTESIAN_POINT('',(-1.56403124237433,1.7,1.75));
#12586=CARTESIAN_POINT('',(-1.56403124237433,1.7,1.7));
#12587=CARTESIAN_POINT('',(-1.71,1.9,1.75));
#12588=CARTESIAN_POINT('Origin',(-1.5,1.9,1.75));
#12589=CARTESIAN_POINT('',(-1.71,1.9,2.4));
#12590=CARTESIAN_POINT('',(-1.71,1.9,1.7));
#12591=CARTESIAN_POINT('Origin',(-1.5,1.9,2.4));
#12592=CARTESIAN_POINT('',(-1.43596875762567,1.7,1.75));
#12593=CARTESIAN_POINT('Origin',(-1.5,1.9,1.75));
#12594=CARTESIAN_POINT('',(-1.43596875762567,1.7,1.7));
#12595=CARTESIAN_POINT('Origin',(-1.5,-1.9,1.7));
#12596=CARTESIAN_POINT('',(-1.43596875762567,-1.7,1.7));
#12597=CARTESIAN_POINT('',(-1.56403124237433,-1.7,1.7));
#12598=CARTESIAN_POINT('',(-0.75,-1.7,1.7));
#12599=CARTESIAN_POINT('Origin',(-1.5,-1.9,1.7));
#12600=CARTESIAN_POINT('Origin',(-1.5,-1.9,1.7));
#12601=CARTESIAN_POINT('',(-1.43596875762567,-1.7,1.75));
#12602=CARTESIAN_POINT('',(-1.43596875762567,-1.7,1.7));
#12603=CARTESIAN_POINT('',(-1.71,-1.9,1.75));
#12604=CARTESIAN_POINT('Origin',(-1.5,-1.9,1.75));
#12605=CARTESIAN_POINT('',(-1.71,-1.9,2.4));
#12606=CARTESIAN_POINT('',(-1.71,-1.9,1.7));
#12607=CARTESIAN_POINT('Origin',(-1.5,-1.9,2.4));
#12608=CARTESIAN_POINT('',(-1.56403124237433,-1.7,1.75));
#12609=CARTESIAN_POINT('Origin',(-1.5,-1.9,1.75));
#12610=CARTESIAN_POINT('',(-1.56403124237433,-1.7,1.7));
#12611=CARTESIAN_POINT('Origin',(1.5,1.9,1.7));
#12612=CARTESIAN_POINT('',(1.43596875762567,1.7,1.7));
#12613=CARTESIAN_POINT('',(1.56403124237433,1.7,1.7));
#12614=CARTESIAN_POINT('',(0.75,1.7,1.7));
#12615=CARTESIAN_POINT('Origin',(1.5,1.9,1.7));
#12616=CARTESIAN_POINT('Origin',(1.5,1.9,1.7));
#12617=CARTESIAN_POINT('',(1.43596875762567,1.7,1.75));
#12618=CARTESIAN_POINT('',(1.43596875762567,1.7,1.7));
#12619=CARTESIAN_POINT('',(1.29,1.9,1.75));
#12620=CARTESIAN_POINT('Origin',(1.5,1.9,1.75));
#12621=CARTESIAN_POINT('',(1.29,1.9,2.4));
#12622=CARTESIAN_POINT('',(1.29,1.9,1.7));
#12623=CARTESIAN_POINT('Origin',(1.5,1.9,2.4));
#12624=CARTESIAN_POINT('',(1.56403124237433,1.7,1.75));
#12625=CARTESIAN_POINT('Origin',(1.5,1.9,1.75));
#12626=CARTESIAN_POINT('',(1.56403124237433,1.7,1.7));
#12627=CARTESIAN_POINT('Origin',(0.,-1.7,1.75));
#12628=CARTESIAN_POINT('',(0.,-1.7,1.75));
#12629=CARTESIAN_POINT('',(-1.97,-1.7,1.75));
#12630=CARTESIAN_POINT('',(0.,-1.7,1.75));
#12631=CARTESIAN_POINT('',(-1.97,-1.7,0.43));
#12632=CARTESIAN_POINT('',(-1.97,-1.7,1.75));
#12633=CARTESIAN_POINT('',(1.97,-1.7,0.43));
#12634=CARTESIAN_POINT('',(0.,-1.7,0.43));
#12635=CARTESIAN_POINT('',(1.97,-1.7,1.75));
#12636=CARTESIAN_POINT('',(1.97,-1.7,1.75));
#12637=CARTESIAN_POINT('',(0.,-1.7,1.75));
#12638=CARTESIAN_POINT('Origin',(0.,1.7,0.43));
#12639=CARTESIAN_POINT('',(0.,1.7,1.75));
#12640=CARTESIAN_POINT('',(1.97,1.7,1.75));
#12641=CARTESIAN_POINT('',(0.,1.7,1.75));
#12642=CARTESIAN_POINT('',(1.97,1.7,0.43));
#12643=CARTESIAN_POINT('',(1.97,1.7,0.43));
#12644=CARTESIAN_POINT('',(-1.97,1.7,0.43));
#12645=CARTESIAN_POINT('',(0.,1.7,0.43));
#12646=CARTESIAN_POINT('',(-1.97,1.7,1.75));
#12647=CARTESIAN_POINT('',(-1.97,1.7,0.43));
#12648=CARTESIAN_POINT('',(0.,1.7,1.75));
#12649=CARTESIAN_POINT('Origin',(-1.97,0.,1.415));
#12650=CARTESIAN_POINT('',(-1.97,-2.35,1.75));
#12651=CARTESIAN_POINT('',(-1.97,-2.35,1.75));
#12652=CARTESIAN_POINT('',(-1.97,-2.35,2.4));
#12653=CARTESIAN_POINT('',(-1.97,-2.35,2.4));
#12654=CARTESIAN_POINT('',(-1.97,2.35,2.4));
#12655=CARTESIAN_POINT('',(-1.97,2.35,2.4));
#12656=CARTESIAN_POINT('',(-1.97,2.35,1.75));
#12657=CARTESIAN_POINT('',(-1.97,2.35,1.75));
#12658=CARTESIAN_POINT('',(-1.97,1.7,1.75));
#12659=CARTESIAN_POINT('',(-1.97,0.78,0.43));
#12660=CARTESIAN_POINT('',(-1.97,0.78,0.43));
#12661=CARTESIAN_POINT('',(-1.97,0.78,1.55));
#12662=CARTESIAN_POINT('',(-1.97,0.78,1.55));
#12663=CARTESIAN_POINT('',(-1.97,-0.78,1.55));
#12664=CARTESIAN_POINT('',(-1.97,-0.78,1.55));
#12665=CARTESIAN_POINT('',(-1.97,-0.78,0.43));
#12666=CARTESIAN_POINT('',(-1.97,-0.78,0.43));
#12667=CARTESIAN_POINT('',(-1.97,-1.7,0.43));
#12668=CARTESIAN_POINT('Origin',(0.,-2.35,1.75));
#12669=CARTESIAN_POINT('',(1.97,-2.35,1.75));
#12670=CARTESIAN_POINT('',(1.97,-2.35,1.75));
#12671=CARTESIAN_POINT('',(0.,-2.35,1.75));
#12672=CARTESIAN_POINT('Origin',(0.,-2.35,2.4));
#12673=CARTESIAN_POINT('',(1.97,-2.35,2.4));
#12674=CARTESIAN_POINT('',(1.97,-2.35,2.4));
#12675=CARTESIAN_POINT('',(0.,-2.35,2.4));
#12676=CARTESIAN_POINT('Origin',(0.,2.35,2.4));
#12677=CARTESIAN_POINT('',(1.97,2.35,2.4));
#12678=CARTESIAN_POINT('',(1.97,2.35,2.4));
#12679=CARTESIAN_POINT('',(0.,2.35,2.4));
#12680=CARTESIAN_POINT('Origin',(0.,2.35,1.75));
#12681=CARTESIAN_POINT('',(1.97,2.35,1.75));
#12682=CARTESIAN_POINT('',(1.97,2.35,1.75));
#12683=CARTESIAN_POINT('',(0.,2.35,1.75));
#12684=CARTESIAN_POINT('Origin',(0.,1.7,1.75));
#12685=CARTESIAN_POINT('',(1.97,1.7,1.75));
#12686=CARTESIAN_POINT('Origin',(0.,0.78,0.43));
#12687=CARTESIAN_POINT('',(1.97,0.78,0.43));
#12688=CARTESIAN_POINT('',(1.97,0.78,0.43));
#12689=CARTESIAN_POINT('',(0.,0.78,0.43));
#12690=CARTESIAN_POINT('Origin',(0.,0.78,1.55));
#12691=CARTESIAN_POINT('',(1.97,0.78,1.55));
#12692=CARTESIAN_POINT('',(1.97,0.78,1.55));
#12693=CARTESIAN_POINT('',(0.,0.78,1.55));
#12694=CARTESIAN_POINT('Origin',(0.,-0.78,1.55));
#12695=CARTESIAN_POINT('',(1.97,-0.78,1.55));
#12696=CARTESIAN_POINT('',(1.97,-0.78,1.55));
#12697=CARTESIAN_POINT('',(0.,-0.78,1.55));
#12698=CARTESIAN_POINT('Origin',(0.,-0.78,0.43));
#12699=CARTESIAN_POINT('',(1.97,-0.78,0.43));
#12700=CARTESIAN_POINT('',(1.97,-0.78,0.43));
#12701=CARTESIAN_POINT('',(0.,-0.78,0.43));
#12702=CARTESIAN_POINT('Origin',(0.,-1.7,0.43));
#12703=CARTESIAN_POINT('',(1.97,-1.7,0.43));
#12704=CARTESIAN_POINT('Origin',(1.97,0.,1.415));
#13052=UNCERTAINTY_MEASURE_WITH_UNIT(LENGTH_MEASURE(0.001),#13095,
'DISTANCE_ACCURACY_VALUE',
'Maximum model space distance between geometric entities at asserted c
onnectivities');
#13057=UNCERTAINTY_MEASURE_WITH_UNIT(LENGTH_MEASURE(0.001),#13095,
'DISTANCE_ACCURACY_VALUE',
'Maximum model space distance between geometric entities at asserted c
onnectivities');
#13089=(
GEOMETRIC_REPRESENTATION_CONTEXT(3)
GLOBAL_UNCERTAINTY_ASSIGNED_CONTEXT((#13052))
GLOBAL_UNIT_ASSIGNED_CONTEXT((#13095,#13097,#13098))
REPRESENTATION_CONTEXT('','3D')
);
#13094=(
GEOMETRIC_REPRESENTATION_CONTEXT(3)
GLOBAL_UNCERTAINTY_ASSIGNED_CONTEXT((#13057))
GLOBAL_UNIT_ASSIGNED_CONTEXT((#13095,#13097,#13098))
REPRESENTATION_CONTEXT('','3D')
);
#13095=(
LENGTH_UNIT()
NAMED_UNIT(*)
SI_UNIT(.CENTI.,.METRE.)
);
#13097=(
NAMED_UNIT(*)
PLANE_ANGLE_UNIT()
SI_UNIT($,.RADIAN.)
);
#13098=(
NAMED_UNIT(*)
SI_UNIT($,.STERADIAN.)
SOLID_ANGLE_UNIT()
);
#13130=SHAPE_DEFINITION_REPRESENTATION(#13166,#13280);
#13166=PRODUCT_DEFINITION_SHAPE('',$,#13317);
#13280=SHAPE_REPRESENTATION('',(#8509),#13089);
#13285=PRODUCT_DEFINITION_CONTEXT('part definition',#13395,'design');
#13317=PRODUCT_DEFINITION('Block','Block',#13353,#13285);
#13353=PRODUCT_DEFINITION_FORMATION('',$,#13428);
#13395=APPLICATION_CONTEXT(
'Core Data for Automotive Mechanical Design Process');
#13396=PRODUCT_CONTEXT('part definition',#13395,'mechanical');
#13428=PRODUCT('Block','Block','Block',(#13396));
#13468=COLOUR_RGB('Dark Blue',0.08,0.2,0.34);
#13469=FILL_AREA_STYLE_COLOUR('',#13468);
#13470=FILL_AREA_STYLE('',(#13469));
#13471=SURFACE_STYLE_FILL_AREA(#13470);
#13472=SURFACE_SIDE_STYLE('',(#13471));
#13473=SURFACE_STYLE_USAGE(.BOTH.,#13472);
#13474=PRESENTATION_STYLE_ASSIGNMENT((#13473));
ENDSEC;
END-ISO-10303-21;
